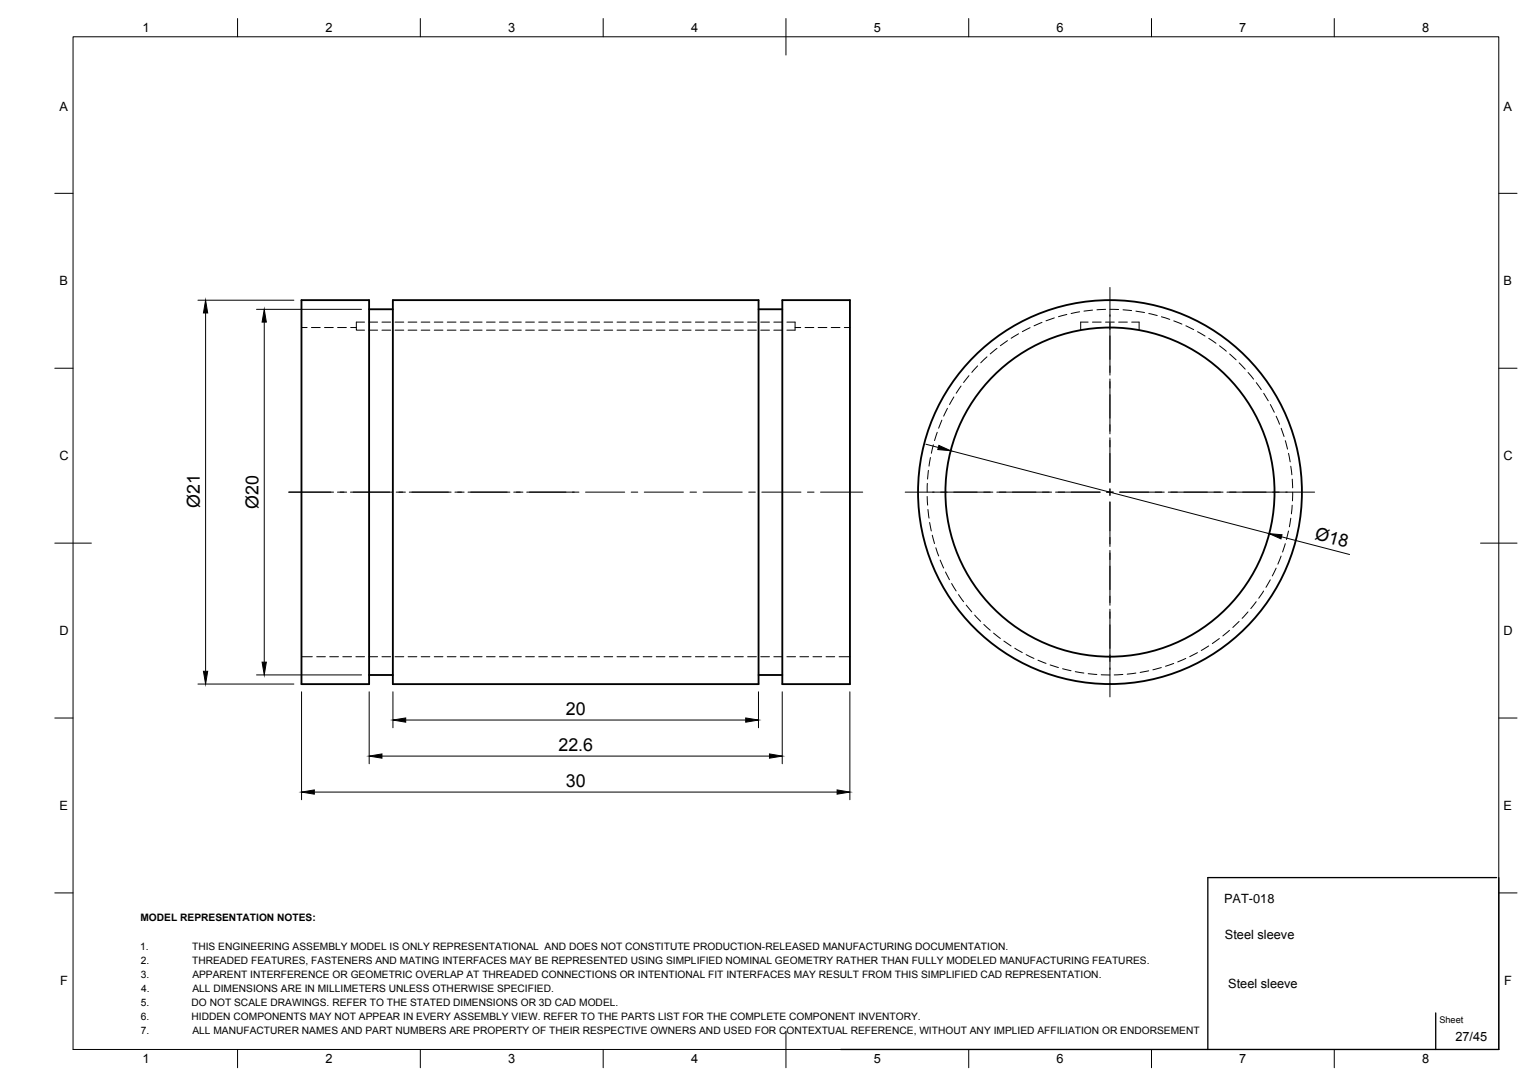
ISO-10303-21;
HEADER;
/* Generated by software containing ST-Developer
 * from STEP Tools, Inc. (www.steptools.com) 
 */

FILE_DESCRIPTION(
/* description */ ('Cam-driven reciprocating slide'),
/* implementation_level */ '2;1');

FILE_NAME(
/* name */ 'Steel sleeve.step',
/* time_stamp */ '2026-10-28T03:25:20-07:00',
/* author */ (''),
/* organization */ (''),
/* preprocessor_version */ 'ST-DEVELOPER v20.2',
/* originating_system */ 'Autodesk Translation Framework v15.17.0.0',
/* authorisation */ '');

FILE_SCHEMA (('AUTOMOTIVE_DESIGN { 1 0 10303 214 3 1 1 }'));
ENDSEC;

DATA;
#10=MECHANICAL_DESIGN_GEOMETRIC_PRESENTATION_REPRESENTATION('',(#448),#13277);
#367=SHAPE_REPRESENTATION_RELATIONSHIP('SRR','None',#13462,#404);
#404=ADVANCED_BREP_SHAPE_REPRESENTATION('',(#491),#13257);
#448=STYLED_ITEM('',(#13734),#491);
#491=MANIFOLD_SOLID_BREP('Body1',#6425);
#628=FACE_BOUND('',#1623,.T.);
#629=FACE_BOUND('',#1626,.T.);
#630=FACE_BOUND('',#1629,.T.);
#631=FACE_BOUND('',#1632,.T.);
#632=FACE_BOUND('',#1635,.T.);
#633=FACE_BOUND('',#1638,.T.);
#634=FACE_BOUND('',#1640,.T.);
#791=PLANE('',#7310);
#792=PLANE('',#7312);
#793=PLANE('',#7313);
#794=PLANE('',#7315);
#795=PLANE('',#7316);
#796=PLANE('',#7317);
#797=PLANE('',#7322);
#798=PLANE('',#7326);
#799=PLANE('',#7330);
#800=PLANE('',#7334);
#801=PLANE('',#7338);
#1117=FACE_OUTER_BOUND('',#1617,.T.);
#1118=FACE_OUTER_BOUND('',#1618,.T.);
#1119=FACE_OUTER_BOUND('',#1619,.T.);
#1120=FACE_OUTER_BOUND('',#1620,.T.);
#1121=FACE_OUTER_BOUND('',#1621,.T.);
#1122=FACE_OUTER_BOUND('',#1622,.T.);
#1123=FACE_OUTER_BOUND('',#1624,.T.);
#1124=FACE_OUTER_BOUND('',#1625,.T.);
#1125=FACE_OUTER_BOUND('',#1627,.T.);
#1126=FACE_OUTER_BOUND('',#1628,.T.);
#1127=FACE_OUTER_BOUND('',#1630,.T.);
#1128=FACE_OUTER_BOUND('',#1631,.T.);
#1129=FACE_OUTER_BOUND('',#1633,.T.);
#1130=FACE_OUTER_BOUND('',#1634,.T.);
#1131=FACE_OUTER_BOUND('',#1636,.T.);
#1132=FACE_OUTER_BOUND('',#1637,.T.);
#1133=FACE_OUTER_BOUND('',#1639,.T.);
#1617=EDGE_LOOP('',(#5270,#5271,#5272,#5273));
#1618=EDGE_LOOP('',(#5274,#5275,#5276,#5277));
#1619=EDGE_LOOP('',(#5278,#5279,#5280,#5281));
#1620=EDGE_LOOP('',(#5282,#5283,#5284,#5285));
#1621=EDGE_LOOP('',(#5286,#5287,#5288,#5289));
#1622=EDGE_LOOP('',(#5290));
#1623=EDGE_LOOP('',(#5291));
#1624=EDGE_LOOP('',(#5292,#5293,#5294,#5295));
#1625=EDGE_LOOP('',(#5296));
#1626=EDGE_LOOP('',(#5297));
#1627=EDGE_LOOP('',(#5298,#5299,#5300,#5301));
#1628=EDGE_LOOP('',(#5302));
#1629=EDGE_LOOP('',(#5303));
#1630=EDGE_LOOP('',(#5304,#5305,#5306,#5307));
#1631=EDGE_LOOP('',(#5308));
#1632=EDGE_LOOP('',(#5309));
#1633=EDGE_LOOP('',(#5310,#5311,#5312,#5313));
#1634=EDGE_LOOP('',(#5314));
#1635=EDGE_LOOP('',(#5315));
#1636=EDGE_LOOP('',(#5316,#5317,#5318,#5319));
#1637=EDGE_LOOP('',(#5320));
#1638=EDGE_LOOP('',(#5321));
#1639=EDGE_LOOP('',(#5322,#5323,#5324,#5325));
#1640=EDGE_LOOP('',(#5326,#5327,#5328,#5329));
#2072=LINE('',#12431,#2511);
#2073=LINE('',#12433,#2512);
#2074=LINE('',#12434,#2513);
#2075=LINE('',#12437,#2514);
#2076=LINE('',#12439,#2515);
#2077=LINE('',#12440,#2516);
#2078=LINE('',#12445,#2517);
#2079=LINE('',#12446,#2518);
#2080=LINE('',#12448,#2519);
#2081=LINE('',#12449,#2520);
#2082=LINE('',#12459,#2521);
#2083=LINE('',#12466,#2522);
#2084=LINE('',#12473,#2523);
#2085=LINE('',#12480,#2524);
#2086=LINE('',#12487,#2525);
#2087=LINE('',#12492,#2526);
#2511=VECTOR('',#8826,1.);
#2512=VECTOR('',#8827,1.);
#2513=VECTOR('',#8828,1.);
#2514=VECTOR('',#8831,1.);
#2515=VECTOR('',#8832,1.);
#2516=VECTOR('',#8833,1.);
#2517=VECTOR('',#8838,1.);
#2518=VECTOR('',#8839,1.);
#2519=VECTOR('',#8842,1.);
#2520=VECTOR('',#8843,1.);
#2521=VECTOR('',#8856,1.05);
#2522=VECTOR('',#8865,1.);
#2523=VECTOR('',#8874,1.05);
#2524=VECTOR('',#8883,1.);
#2525=VECTOR('',#8892,1.05);
#2526=VECTOR('',#8899,0.9);
#2924=CIRCLE('',#7311,0.9);
#2925=CIRCLE('',#7314,0.9);
#2926=CIRCLE('',#7318,1.05);
#2927=CIRCLE('',#7319,0.9);
#2928=CIRCLE('',#7321,1.05);
#2929=CIRCLE('',#7323,1.);
#2930=CIRCLE('',#7325,1.);
#2931=CIRCLE('',#7327,1.05);
#2932=CIRCLE('',#7329,1.05);
#2933=CIRCLE('',#7331,1.);
#2934=CIRCLE('',#7333,1.);
#2935=CIRCLE('',#7335,1.05);
#2936=CIRCLE('',#7337,1.05);
#2937=CIRCLE('',#7339,0.9);
#3353=VERTEX_POINT('',#12427);
#3354=VERTEX_POINT('',#12428);
#3355=VERTEX_POINT('',#12430);
#3356=VERTEX_POINT('',#12432);
#3357=VERTEX_POINT('',#12436);
#3358=VERTEX_POINT('',#12438);
#3359=VERTEX_POINT('',#12442);
#3360=VERTEX_POINT('',#12444);
#3361=VERTEX_POINT('',#12452);
#3362=VERTEX_POINT('',#12454);
#3363=VERTEX_POINT('',#12457);
#3364=VERTEX_POINT('',#12461);
#3365=VERTEX_POINT('',#12464);
#3366=VERTEX_POINT('',#12468);
#3367=VERTEX_POINT('',#12471);
#3368=VERTEX_POINT('',#12475);
#3369=VERTEX_POINT('',#12478);
#3370=VERTEX_POINT('',#12482);
#3371=VERTEX_POINT('',#12485);
#3372=VERTEX_POINT('',#12489);
#4025=EDGE_CURVE('',#3353,#3354,#2924,.T.);
#4026=EDGE_CURVE('',#3355,#3353,#2072,.T.);
#4027=EDGE_CURVE('',#3356,#3355,#2073,.T.);
#4028=EDGE_CURVE('',#3354,#3356,#2074,.T.);
#4029=EDGE_CURVE('',#3354,#3357,#2075,.T.);
#4030=EDGE_CURVE('',#3358,#3356,#2076,.T.);
#4031=EDGE_CURVE('',#3358,#3357,#2077,.T.);
#4032=EDGE_CURVE('',#3357,#3359,#2925,.T.);
#4033=EDGE_CURVE('',#3360,#3358,#2078,.T.);
#4034=EDGE_CURVE('',#3359,#3360,#2079,.T.);
#4035=EDGE_CURVE('',#3359,#3353,#2080,.T.);
#4036=EDGE_CURVE('',#3360,#3355,#2081,.T.);
#4037=EDGE_CURVE('',#3361,#3361,#2926,.T.);
#4038=EDGE_CURVE('',#3362,#3362,#2927,.T.);
#4039=EDGE_CURVE('',#3363,#3363,#2928,.T.);
#4040=EDGE_CURVE('',#3363,#3361,#2082,.T.);
#4041=EDGE_CURVE('',#3364,#3364,#2929,.T.);
#4042=EDGE_CURVE('',#3365,#3365,#2930,.T.);
#4043=EDGE_CURVE('',#3365,#3364,#2083,.T.);
#4044=EDGE_CURVE('',#3366,#3366,#2931,.T.);
#4045=EDGE_CURVE('',#3367,#3367,#2932,.T.);
#4046=EDGE_CURVE('',#3367,#3366,#2084,.T.);
#4047=EDGE_CURVE('',#3368,#3368,#2933,.T.);
#4048=EDGE_CURVE('',#3369,#3369,#2934,.T.);
#4049=EDGE_CURVE('',#3369,#3368,#2085,.T.);
#4050=EDGE_CURVE('',#3370,#3370,#2935,.T.);
#4051=EDGE_CURVE('',#3371,#3371,#2936,.T.);
#4052=EDGE_CURVE('',#3371,#3370,#2086,.T.);
#4053=EDGE_CURVE('',#3372,#3372,#2937,.T.);
#4054=EDGE_CURVE('',#3372,#3362,#2087,.T.);
#5270=ORIENTED_EDGE('',*,*,#4025,.F.);
#5271=ORIENTED_EDGE('',*,*,#4026,.F.);
#5272=ORIENTED_EDGE('',*,*,#4027,.F.);
#5273=ORIENTED_EDGE('',*,*,#4028,.F.);
#5274=ORIENTED_EDGE('',*,*,#4029,.F.);
#5275=ORIENTED_EDGE('',*,*,#4028,.T.);
#5276=ORIENTED_EDGE('',*,*,#4030,.F.);
#5277=ORIENTED_EDGE('',*,*,#4031,.T.);
#5278=ORIENTED_EDGE('',*,*,#4032,.F.);
#5279=ORIENTED_EDGE('',*,*,#4031,.F.);
#5280=ORIENTED_EDGE('',*,*,#4033,.F.);
#5281=ORIENTED_EDGE('',*,*,#4034,.F.);
#5282=ORIENTED_EDGE('',*,*,#4035,.F.);
#5283=ORIENTED_EDGE('',*,*,#4034,.T.);
#5284=ORIENTED_EDGE('',*,*,#4036,.T.);
#5285=ORIENTED_EDGE('',*,*,#4026,.T.);
#5286=ORIENTED_EDGE('',*,*,#4036,.F.);
#5287=ORIENTED_EDGE('',*,*,#4033,.T.);
#5288=ORIENTED_EDGE('',*,*,#4030,.T.);
#5289=ORIENTED_EDGE('',*,*,#4027,.T.);
#5290=ORIENTED_EDGE('',*,*,#4037,.F.);
#5291=ORIENTED_EDGE('',*,*,#4038,.T.);
#5292=ORIENTED_EDGE('',*,*,#4039,.F.);
#5293=ORIENTED_EDGE('',*,*,#4040,.T.);
#5294=ORIENTED_EDGE('',*,*,#4037,.T.);
#5295=ORIENTED_EDGE('',*,*,#4040,.F.);
#5296=ORIENTED_EDGE('',*,*,#4039,.T.);
#5297=ORIENTED_EDGE('',*,*,#4041,.F.);
#5298=ORIENTED_EDGE('',*,*,#4042,.F.);
#5299=ORIENTED_EDGE('',*,*,#4043,.T.);
#5300=ORIENTED_EDGE('',*,*,#4041,.T.);
#5301=ORIENTED_EDGE('',*,*,#4043,.F.);
#5302=ORIENTED_EDGE('',*,*,#4044,.F.);
#5303=ORIENTED_EDGE('',*,*,#4042,.T.);
#5304=ORIENTED_EDGE('',*,*,#4045,.F.);
#5305=ORIENTED_EDGE('',*,*,#4046,.T.);
#5306=ORIENTED_EDGE('',*,*,#4044,.T.);
#5307=ORIENTED_EDGE('',*,*,#4046,.F.);
#5308=ORIENTED_EDGE('',*,*,#4045,.T.);
#5309=ORIENTED_EDGE('',*,*,#4047,.F.);
#5310=ORIENTED_EDGE('',*,*,#4048,.F.);
#5311=ORIENTED_EDGE('',*,*,#4049,.T.);
#5312=ORIENTED_EDGE('',*,*,#4047,.T.);
#5313=ORIENTED_EDGE('',*,*,#4049,.F.);
#5314=ORIENTED_EDGE('',*,*,#4050,.F.);
#5315=ORIENTED_EDGE('',*,*,#4048,.T.);
#5316=ORIENTED_EDGE('',*,*,#4051,.F.);
#5317=ORIENTED_EDGE('',*,*,#4052,.T.);
#5318=ORIENTED_EDGE('',*,*,#4050,.T.);
#5319=ORIENTED_EDGE('',*,*,#4052,.F.);
#5320=ORIENTED_EDGE('',*,*,#4051,.T.);
#5321=ORIENTED_EDGE('',*,*,#4053,.F.);
#5322=ORIENTED_EDGE('',*,*,#4053,.T.);
#5323=ORIENTED_EDGE('',*,*,#4054,.T.);
#5324=ORIENTED_EDGE('',*,*,#4038,.F.);
#5325=ORIENTED_EDGE('',*,*,#4054,.F.);
#5326=ORIENTED_EDGE('',*,*,#4032,.T.);
#5327=ORIENTED_EDGE('',*,*,#4035,.T.);
#5328=ORIENTED_EDGE('',*,*,#4025,.T.);
#5329=ORIENTED_EDGE('',*,*,#4029,.T.);
#5973=CYLINDRICAL_SURFACE('',#7320,1.05);
#5974=CYLINDRICAL_SURFACE('',#7324,1.);
#5975=CYLINDRICAL_SURFACE('',#7328,1.05);
#5976=CYLINDRICAL_SURFACE('',#7332,1.);
#5977=CYLINDRICAL_SURFACE('',#7336,1.05);
#5978=CYLINDRICAL_SURFACE('',#7340,0.9);
#6235=ADVANCED_FACE('',(#1117),#791,.F.);
#6236=ADVANCED_FACE('',(#1118),#792,.F.);
#6237=ADVANCED_FACE('',(#1119),#793,.F.);
#6238=ADVANCED_FACE('',(#1120),#794,.F.);
#6239=ADVANCED_FACE('',(#1121),#795,.F.);
#6240=ADVANCED_FACE('',(#1122,#628),#796,.T.);
#6241=ADVANCED_FACE('',(#1123),#5973,.T.);
#6242=ADVANCED_FACE('',(#1124,#629),#797,.T.);
#6243=ADVANCED_FACE('',(#1125),#5974,.T.);
#6244=ADVANCED_FACE('',(#1126,#630),#798,.T.);
#6245=ADVANCED_FACE('',(#1127),#5975,.T.);
#6246=ADVANCED_FACE('',(#1128,#631),#799,.T.);
#6247=ADVANCED_FACE('',(#1129),#5976,.T.);
#6248=ADVANCED_FACE('',(#1130,#632),#800,.T.);
#6249=ADVANCED_FACE('',(#1131),#5977,.T.);
#6250=ADVANCED_FACE('',(#1132,#633),#801,.T.);
#6251=ADVANCED_FACE('',(#1133,#634),#5978,.F.);
#6425=CLOSED_SHELL('',(#6235,#6236,#6237,#6238,#6239,#6240,#6241,#6242,
#6243,#6244,#6245,#6246,#6247,#6248,#6249,#6250,#6251));
#7309=AXIS2_PLACEMENT_3D('',#12425,#8820,#8821);
#7310=AXIS2_PLACEMENT_3D('',#12426,#8822,#8823);
#7311=AXIS2_PLACEMENT_3D('',#12429,#8824,#8825);
#7312=AXIS2_PLACEMENT_3D('',#12435,#8829,#8830);
#7313=AXIS2_PLACEMENT_3D('',#12441,#8834,#8835);
#7314=AXIS2_PLACEMENT_3D('',#12443,#8836,#8837);
#7315=AXIS2_PLACEMENT_3D('',#12447,#8840,#8841);
#7316=AXIS2_PLACEMENT_3D('',#12450,#8844,#8845);
#7317=AXIS2_PLACEMENT_3D('',#12451,#8846,#8847);
#7318=AXIS2_PLACEMENT_3D('',#12453,#8848,#8849);
#7319=AXIS2_PLACEMENT_3D('',#12455,#8850,#8851);
#7320=AXIS2_PLACEMENT_3D('',#12456,#8852,#8853);
#7321=AXIS2_PLACEMENT_3D('',#12458,#8854,#8855);
#7322=AXIS2_PLACEMENT_3D('',#12460,#8857,#8858);
#7323=AXIS2_PLACEMENT_3D('',#12462,#8859,#8860);
#7324=AXIS2_PLACEMENT_3D('',#12463,#8861,#8862);
#7325=AXIS2_PLACEMENT_3D('',#12465,#8863,#8864);
#7326=AXIS2_PLACEMENT_3D('',#12467,#8866,#8867);
#7327=AXIS2_PLACEMENT_3D('',#12469,#8868,#8869);
#7328=AXIS2_PLACEMENT_3D('',#12470,#8870,#8871);
#7329=AXIS2_PLACEMENT_3D('',#12472,#8872,#8873);
#7330=AXIS2_PLACEMENT_3D('',#12474,#8875,#8876);
#7331=AXIS2_PLACEMENT_3D('',#12476,#8877,#8878);
#7332=AXIS2_PLACEMENT_3D('',#12477,#8879,#8880);
#7333=AXIS2_PLACEMENT_3D('',#12479,#8881,#8882);
#7334=AXIS2_PLACEMENT_3D('',#12481,#8884,#8885);
#7335=AXIS2_PLACEMENT_3D('',#12483,#8886,#8887);
#7336=AXIS2_PLACEMENT_3D('',#12484,#8888,#8889);
#7337=AXIS2_PLACEMENT_3D('',#12486,#8890,#8891);
#7338=AXIS2_PLACEMENT_3D('',#12488,#8893,#8894);
#7339=AXIS2_PLACEMENT_3D('',#12490,#8895,#8896);
#7340=AXIS2_PLACEMENT_3D('',#12491,#8897,#8898);
#8820=DIRECTION('axis',(0.,0.,1.));
#8821=DIRECTION('refdir',(1.,0.,0.));
#8822=DIRECTION('center_axis',(0.,1.,0.));
#8823=DIRECTION('ref_axis',(0.,0.,1.));
#8824=DIRECTION('center_axis',(0.,-1.,0.));
#8825=DIRECTION('ref_axis',(1.,0.,0.));
#8826=DIRECTION('',(-1.,0.,0.));
#8827=DIRECTION('',(0.,0.,-1.));
#8828=DIRECTION('',(1.,0.,0.));
#8829=DIRECTION('center_axis',(0.,0.,1.));
#8830=DIRECTION('ref_axis',(1.,0.,0.));
#8831=DIRECTION('',(0.,-1.,0.));
#8832=DIRECTION('',(0.,1.,0.));
#8833=DIRECTION('',(-1.,0.,0.));
#8834=DIRECTION('center_axis',(0.,-1.,0.));
#8835=DIRECTION('ref_axis',(0.,0.,-1.));
#8836=DIRECTION('center_axis',(0.,1.,0.));
#8837=DIRECTION('ref_axis',(1.,0.,0.));
#8838=DIRECTION('',(0.,0.,1.));
#8839=DIRECTION('',(1.,0.,0.));
#8840=DIRECTION('center_axis',(0.,0.,-1.));
#8841=DIRECTION('ref_axis',(-1.,0.,0.));
#8842=DIRECTION('',(0.,1.,0.));
#8843=DIRECTION('',(0.,1.,0.));
#8844=DIRECTION('center_axis',(1.,0.,0.));
#8845=DIRECTION('ref_axis',(0.,0.,-1.));
#8846=DIRECTION('center_axis',(0.,1.,0.));
#8847=DIRECTION('ref_axis',(0.,0.,1.));
#8848=DIRECTION('center_axis',(0.,-1.,0.));
#8849=DIRECTION('ref_axis',(1.,0.,0.));
#8850=DIRECTION('center_axis',(0.,-1.,0.));
#8851=DIRECTION('ref_axis',(1.,0.,0.));
#8852=DIRECTION('center_axis',(0.,-1.,0.));
#8853=DIRECTION('ref_axis',(1.,0.,0.));
#8854=DIRECTION('center_axis',(0.,-1.,0.));
#8855=DIRECTION('ref_axis',(1.,0.,0.));
#8856=DIRECTION('',(0.,1.,0.));
#8857=DIRECTION('center_axis',(0.,-1.,0.));
#8858=DIRECTION('ref_axis',(0.,0.,-1.));
#8859=DIRECTION('center_axis',(0.,-1.,0.));
#8860=DIRECTION('ref_axis',(1.,0.,0.));
#8861=DIRECTION('center_axis',(0.,-1.,0.));
#8862=DIRECTION('ref_axis',(1.,0.,0.));
#8863=DIRECTION('center_axis',(0.,-1.,0.));
#8864=DIRECTION('ref_axis',(1.,0.,0.));
#8865=DIRECTION('',(0.,1.,0.));
#8866=DIRECTION('center_axis',(0.,1.,0.));
#8867=DIRECTION('ref_axis',(0.,0.,1.));
#8868=DIRECTION('center_axis',(0.,-1.,0.));
#8869=DIRECTION('ref_axis',(1.,0.,0.));
#8870=DIRECTION('center_axis',(0.,-1.,0.));
#8871=DIRECTION('ref_axis',(1.,0.,0.));
#8872=DIRECTION('center_axis',(0.,-1.,0.));
#8873=DIRECTION('ref_axis',(1.,0.,0.));
#8874=DIRECTION('',(0.,1.,0.));
#8875=DIRECTION('center_axis',(0.,-1.,0.));
#8876=DIRECTION('ref_axis',(0.,0.,-1.));
#8877=DIRECTION('center_axis',(0.,-1.,0.));
#8878=DIRECTION('ref_axis',(1.,0.,0.));
#8879=DIRECTION('center_axis',(0.,-1.,0.));
#8880=DIRECTION('ref_axis',(1.,0.,0.));
#8881=DIRECTION('center_axis',(0.,-1.,0.));
#8882=DIRECTION('ref_axis',(1.,0.,0.));
#8883=DIRECTION('',(0.,1.,0.));
#8884=DIRECTION('center_axis',(0.,1.,0.));
#8885=DIRECTION('ref_axis',(0.,0.,1.));
#8886=DIRECTION('center_axis',(0.,-1.,0.));
#8887=DIRECTION('ref_axis',(1.,0.,0.));
#8888=DIRECTION('center_axis',(0.,-1.,0.));
#8889=DIRECTION('ref_axis',(1.,0.,0.));
#8890=DIRECTION('center_axis',(0.,-1.,0.));
#8891=DIRECTION('ref_axis',(1.,0.,0.));
#8892=DIRECTION('',(0.,1.,0.));
#8893=DIRECTION('center_axis',(0.,-1.,0.));
#8894=DIRECTION('ref_axis',(0.,0.,-1.));
#8895=DIRECTION('center_axis',(0.,-1.,0.));
#8896=DIRECTION('ref_axis',(1.,0.,0.));
#8897=DIRECTION('center_axis',(0.,-1.,0.));
#8898=DIRECTION('ref_axis',(1.,0.,0.));
#8899=DIRECTION('',(0.,1.,0.));
#12425=CARTESIAN_POINT('',(0.,0.,0.));
#12426=CARTESIAN_POINT('Origin',(0.75,1.2,0.));
#12427=CARTESIAN_POINT('',(0.885663593019381,1.2,-0.16));
#12428=CARTESIAN_POINT('',(0.885663593019381,1.2,0.16));
#12429=CARTESIAN_POINT('Origin',(0.,1.2,0.));
#12430=CARTESIAN_POINT('',(0.93,1.2,-0.16));
#12431=CARTESIAN_POINT('',(0.93,1.2,-0.16));
#12432=CARTESIAN_POINT('',(0.93,1.2,0.16));
#12433=CARTESIAN_POINT('',(0.93,1.2,0.16));
#12434=CARTESIAN_POINT('',(0.57,1.2,0.16));
#12435=CARTESIAN_POINT('Origin',(0.57,0.,0.16));
#12436=CARTESIAN_POINT('',(0.885663593019381,-1.2,0.16));
#12437=CARTESIAN_POINT('',(0.885663593019381,0.,0.16));
#12438=CARTESIAN_POINT('',(0.93,-1.2,0.16));
#12439=CARTESIAN_POINT('',(0.93,0.,0.16));
#12440=CARTESIAN_POINT('',(0.57,-1.2,0.16));
#12441=CARTESIAN_POINT('Origin',(0.75,-1.2,0.));
#12442=CARTESIAN_POINT('',(0.885663593019381,-1.2,-0.16));
#12443=CARTESIAN_POINT('Origin',(0.,-1.2,0.));
#12444=CARTESIAN_POINT('',(0.93,-1.2,-0.16));
#12445=CARTESIAN_POINT('',(0.93,-1.2,0.16));
#12446=CARTESIAN_POINT('',(0.93,-1.2,-0.16));
#12447=CARTESIAN_POINT('Origin',(0.93,0.,-0.16));
#12448=CARTESIAN_POINT('',(0.885663593019381,0.,-0.16));
#12449=CARTESIAN_POINT('',(0.93,0.,-0.16));
#12450=CARTESIAN_POINT('Origin',(0.93,0.,0.16));
#12451=CARTESIAN_POINT('Origin',(1.05,1.5,0.));
#12452=CARTESIAN_POINT('',(-1.05,1.5,-1.28587913910472E-16));
#12453=CARTESIAN_POINT('Origin',(0.,1.5,0.));
#12454=CARTESIAN_POINT('',(-0.9,1.5,-1.10218211923262E-16));
#12455=CARTESIAN_POINT('Origin',(0.,1.5,0.));
#12456=CARTESIAN_POINT('Origin',(0.,1.315,0.));
#12457=CARTESIAN_POINT('',(-1.05,1.13,-1.28587913910472E-16));
#12458=CARTESIAN_POINT('Origin',(0.,1.13,0.));
#12459=CARTESIAN_POINT('',(-1.05,1.315,-1.28587913910472E-16));
#12460=CARTESIAN_POINT('Origin',(1.,1.13,0.));
#12461=CARTESIAN_POINT('',(-1.,1.13,-1.22464679914735E-16));
#12462=CARTESIAN_POINT('Origin',(0.,1.13,0.));
#12463=CARTESIAN_POINT('Origin',(0.,1.065,0.));
#12464=CARTESIAN_POINT('',(-1.,1.,-1.22464679914735E-16));
#12465=CARTESIAN_POINT('Origin',(0.,1.,0.));
#12466=CARTESIAN_POINT('',(-1.,1.065,-1.22464679914735E-16));
#12467=CARTESIAN_POINT('Origin',(1.05,1.,0.));
#12468=CARTESIAN_POINT('',(-1.05,1.,-1.28587913910472E-16));
#12469=CARTESIAN_POINT('Origin',(0.,1.,0.));
#12470=CARTESIAN_POINT('Origin',(0.,0.,0.));
#12471=CARTESIAN_POINT('',(-1.05,-1.,-1.28587913910472E-16));
#12472=CARTESIAN_POINT('Origin',(0.,-1.,0.));
#12473=CARTESIAN_POINT('',(-1.05,0.,-1.28587913910472E-16));
#12474=CARTESIAN_POINT('Origin',(1.,-1.,0.));
#12475=CARTESIAN_POINT('',(-1.,-1.,-1.22464679914735E-16));
#12476=CARTESIAN_POINT('Origin',(0.,-1.,0.));
#12477=CARTESIAN_POINT('Origin',(0.,-1.065,0.));
#12478=CARTESIAN_POINT('',(-1.,-1.13,-1.22464679914735E-16));
#12479=CARTESIAN_POINT('Origin',(0.,-1.13,0.));
#12480=CARTESIAN_POINT('',(-1.,-1.065,-1.22464679914735E-16));
#12481=CARTESIAN_POINT('Origin',(1.05,-1.13,0.));
#12482=CARTESIAN_POINT('',(-1.05,-1.13,-1.28587913910472E-16));
#12483=CARTESIAN_POINT('Origin',(0.,-1.13,0.));
#12484=CARTESIAN_POINT('Origin',(0.,-1.315,0.));
#12485=CARTESIAN_POINT('',(-1.05,-1.5,-1.28587913910472E-16));
#12486=CARTESIAN_POINT('Origin',(0.,-1.5,0.));
#12487=CARTESIAN_POINT('',(-1.05,-1.315,-1.28587913910472E-16));
#12488=CARTESIAN_POINT('Origin',(0.9,-1.5,0.));
#12489=CARTESIAN_POINT('',(-0.9,-1.5,-1.10218211923262E-16));
#12490=CARTESIAN_POINT('Origin',(0.,-1.5,0.));
#12491=CARTESIAN_POINT('Origin',(0.,0.,0.));
#12492=CARTESIAN_POINT('',(-0.9,0.,-1.10218211923262E-16));
#13213=UNCERTAINTY_MEASURE_WITH_UNIT(LENGTH_MEASURE(0.001),#13278,
'DISTANCE_ACCURACY_VALUE',
'Maximum model space distance between geometric entities at asserted c
onnectivities');
#13233=UNCERTAINTY_MEASURE_WITH_UNIT(LENGTH_MEASURE(0.001),#13278,
'DISTANCE_ACCURACY_VALUE',
'Maximum model space distance between geometric entities at asserted c
onnectivities');
#13257=(
GEOMETRIC_REPRESENTATION_CONTEXT(3)
GLOBAL_UNCERTAINTY_ASSIGNED_CONTEXT((#13213))
GLOBAL_UNIT_ASSIGNED_CONTEXT((#13278,#13280,#13281))
REPRESENTATION_CONTEXT('','3D')
);
#13277=(
GEOMETRIC_REPRESENTATION_CONTEXT(3)
GLOBAL_UNCERTAINTY_ASSIGNED_CONTEXT((#13233))
GLOBAL_UNIT_ASSIGNED_CONTEXT((#13278,#13280,#13281))
REPRESENTATION_CONTEXT('','3D')
);
#13278=(
LENGTH_UNIT()
NAMED_UNIT(*)
SI_UNIT(.CENTI.,.METRE.)
);
#13280=(
NAMED_UNIT(*)
PLANE_ANGLE_UNIT()
SI_UNIT($,.RADIAN.)
);
#13281=(
NAMED_UNIT(*)
SI_UNIT($,.STERADIAN.)
SOLID_ANGLE_UNIT()
);
#13305=SHAPE_DEFINITION_REPRESENTATION(#13353,#13462);
#13353=PRODUCT_DEFINITION_SHAPE('',$,#13506);
#13462=SHAPE_REPRESENTATION('',(#7309),#13257);
#13482=PRODUCT_DEFINITION_CONTEXT('part definition',#13613,'design');
#13506=PRODUCT_DEFINITION('Steel sleeve','Steel sleeve',#13549,#13482);
#13549=PRODUCT_DEFINITION_FORMATION('',$,#13638);
#13613=APPLICATION_CONTEXT(
'Core Data for Automotive Mechanical Design Process');
#13614=PRODUCT_CONTEXT('part definition',#13613,'mechanical');
#13638=PRODUCT('Steel sleeve','Steel sleeve','Steel sleeve',(#13614));
#13728=COLOUR_RGB('Off White',0.89,0.88,0.83);
#13729=FILL_AREA_STYLE_COLOUR('',#13728);
#13730=FILL_AREA_STYLE('',(#13729));
#13731=SURFACE_STYLE_FILL_AREA(#13730);
#13732=SURFACE_SIDE_STYLE('',(#13731));
#13733=SURFACE_STYLE_USAGE(.BOTH.,#13732);
#13734=PRESENTATION_STYLE_ASSIGNMENT((#13733));
ENDSEC;
END-ISO-10303-21;
